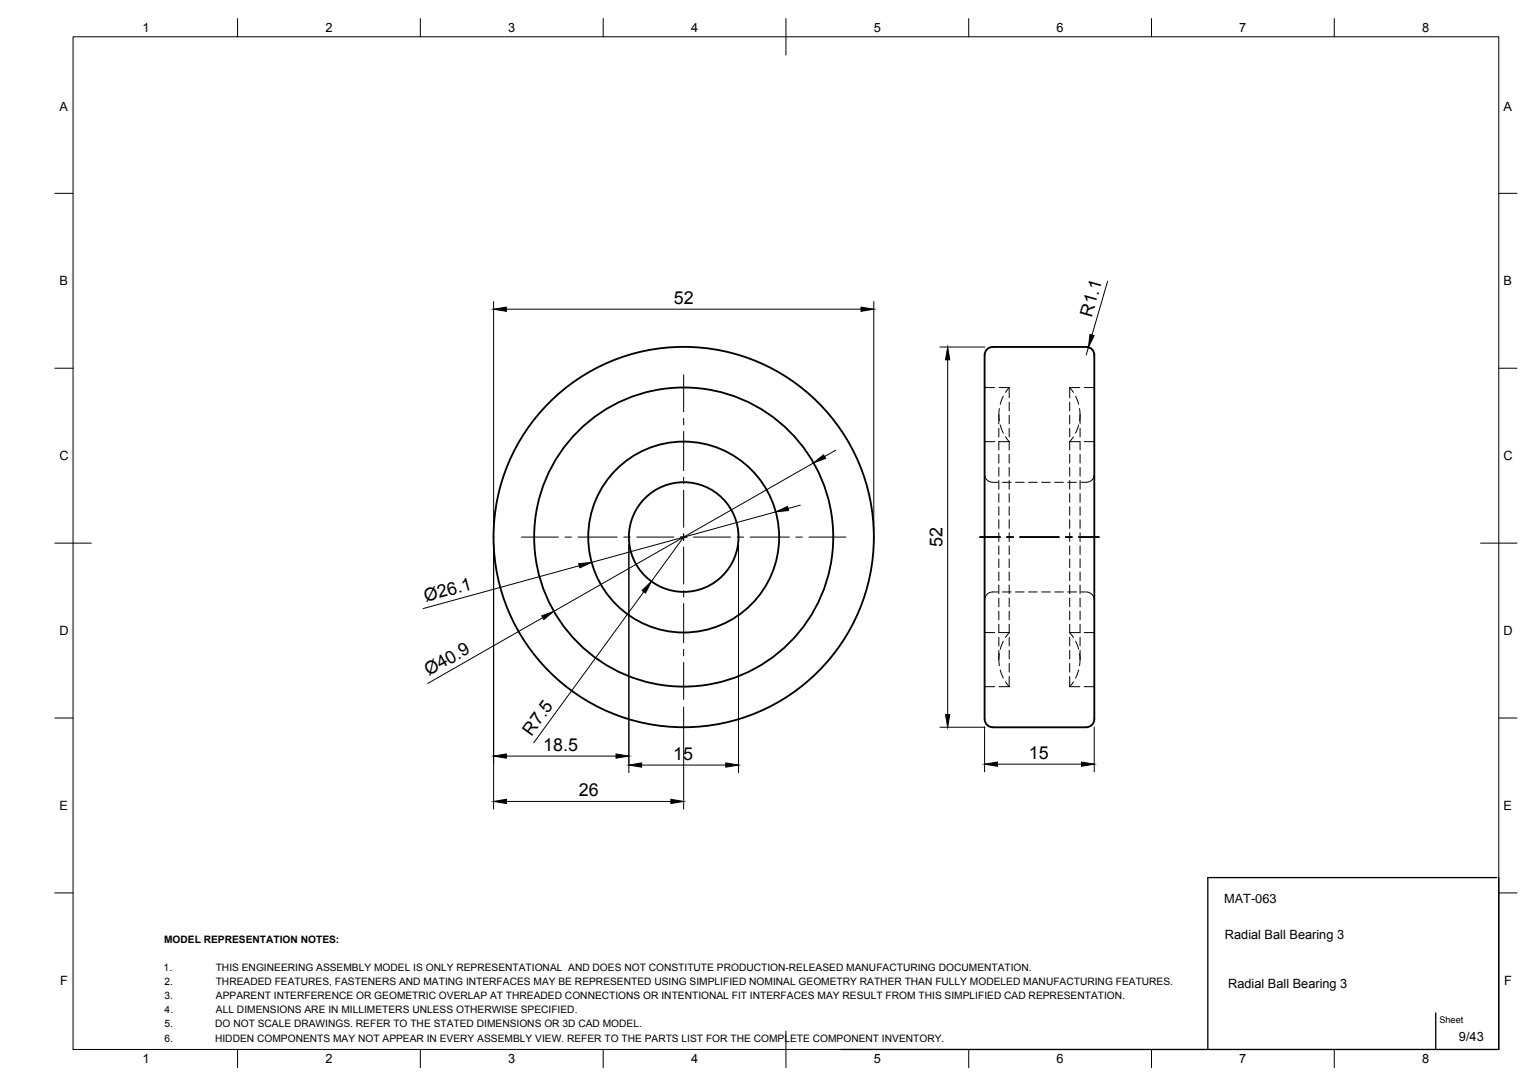
ISO-10303-21;
HEADER;
/* Generated by software containing ST-Developer
 * from STEP Tools, Inc. (www.steptools.com) 
 */

FILE_DESCRIPTION(
/* description */ (''),
/* implementation_level */ '2;1');

FILE_NAME(
/* name */ 'Radial Ball Bearing 3.step',
/* time_stamp */ '2026-10-24T09:43:01-07:00',
/* author */ (''),
/* organization */ (''),
/* preprocessor_version */ 'ST-DEVELOPER v20.2',
/* originating_system */ 'Autodesk Translation Framework v15.15.0.0',
/* authorisation */ '');

FILE_SCHEMA (('AUTOMOTIVE_DESIGN { 1 0 10303 214 3 1 1 }'));
ENDSEC;

DATA;
#10=MECHANICAL_DESIGN_GEOMETRIC_PRESENTATION_REPRESENTATION('',(#279),#11112);
#187=TOROIDAL_SURFACE('',#6680,0.0248999989285722,0.00110000131901909);
#188=TOROIDAL_SURFACE('',#6685,0.0248999989285722,0.00110000131901909);
#189=TOROIDAL_SURFACE('',#6693,0.0248999989285722,0.00110000131901911);
#190=TOROIDAL_SURFACE('',#6700,0.0248999989285722,0.00110000131901911);
#191=TOROIDAL_SURFACE('',#6704,0.01675,0.00555000054498457);
#192=TOROIDAL_SURFACE('',#6713,0.01675,0.00555000054498457);
#193=TOROIDAL_SURFACE('',#6722,0.00860000107142784,0.00110000131901912);
#194=TOROIDAL_SURFACE('',#6726,0.00860000107142784,0.00110000131901912);
#195=TOROIDAL_SURFACE('',#6734,0.00860000107142785,0.00110000131901912);
#196=TOROIDAL_SURFACE('',#6737,0.00860000107142785,0.00110000131901912);
#213=SHAPE_REPRESENTATION_RELATIONSHIP('SRR','None',#11236,#246);
#246=ADVANCED_BREP_SHAPE_REPRESENTATION('',(#312),#11081);
#279=STYLED_ITEM('',(#11425),#312);
#312=MANIFOLD_SOLID_BREP('Radial Ball Bearing 3',#6016);
#393=FACE_BOUND('',#1206,.T.);
#394=FACE_BOUND('',#1211,.T.);
#395=FACE_BOUND('',#1217,.T.);
#396=FACE_BOUND('',#1222,.T.);
#530=PLANE('',#6691);
#531=PLANE('',#6702);
#532=PLANE('',#6717);
#533=PLANE('',#6728);
#784=FACE_OUTER_BOUND('',#1202,.T.);
#785=FACE_OUTER_BOUND('',#1203,.T.);
#786=FACE_OUTER_BOUND('',#1204,.T.);
#787=FACE_OUTER_BOUND('',#1205,.T.);
#788=FACE_OUTER_BOUND('',#1207,.T.);
#789=FACE_OUTER_BOUND('',#1208,.T.);
#790=FACE_OUTER_BOUND('',#1209,.T.);
#791=FACE_OUTER_BOUND('',#1210,.T.);
#792=FACE_OUTER_BOUND('',#1212,.T.);
#793=FACE_OUTER_BOUND('',#1213,.T.);
#794=FACE_OUTER_BOUND('',#1214,.T.);
#795=FACE_OUTER_BOUND('',#1215,.T.);
#796=FACE_OUTER_BOUND('',#1216,.T.);
#797=FACE_OUTER_BOUND('',#1218,.T.);
#798=FACE_OUTER_BOUND('',#1219,.T.);
#799=FACE_OUTER_BOUND('',#1220,.T.);
#800=FACE_OUTER_BOUND('',#1221,.T.);
#801=FACE_OUTER_BOUND('',#1223,.T.);
#802=FACE_OUTER_BOUND('',#1224,.T.);
#803=FACE_OUTER_BOUND('',#1225,.T.);
#1202=EDGE_LOOP('',(#4431,#4432,#4433,#4434));
#1203=EDGE_LOOP('',(#4435,#4436,#4437,#4438));
#1204=EDGE_LOOP('',(#4439,#4440,#4441,#4442,#4443,#4444));
#1205=EDGE_LOOP('',(#4445,#4446));
#1206=EDGE_LOOP('',(#4447));
#1207=EDGE_LOOP('',(#4448,#4449,#4450,#4451));
#1208=EDGE_LOOP('',(#4452,#4453,#4454,#4455,#4456));
#1209=EDGE_LOOP('',(#4457,#4458,#4459,#4460));
#1210=EDGE_LOOP('',(#4461,#4462));
#1211=EDGE_LOOP('',(#4463));
#1212=EDGE_LOOP('',(#4464,#4465,#4466,#4467,#4468,#4469));
#1213=EDGE_LOOP('',(#4470,#4471,#4472,#4473,#4474));
#1214=EDGE_LOOP('',(#4475,#4476,#4477,#4478,#4479));
#1215=EDGE_LOOP('',(#4480,#4481,#4482,#4483,#4484,#4485));
#1216=EDGE_LOOP('',(#4486));
#1217=EDGE_LOOP('',(#4487,#4488));
#1218=EDGE_LOOP('',(#4489,#4490,#4491,#4492,#4493));
#1219=EDGE_LOOP('',(#4494,#4495,#4496,#4497));
#1220=EDGE_LOOP('',(#4498,#4499,#4500,#4501));
#1221=EDGE_LOOP('',(#4502));
#1222=EDGE_LOOP('',(#4503,#4504));
#1223=EDGE_LOOP('',(#4505,#4506,#4507,#4508,#4509,#4510));
#1224=EDGE_LOOP('',(#4511,#4512,#4513,#4514));
#1225=EDGE_LOOP('',(#4515,#4516,#4517,#4518));
#1643=LINE('',#9850,#2002);
#1644=LINE('',#9862,#2003);
#1645=LINE('',#9882,#2004);
#1646=LINE('',#9885,#2005);
#1647=LINE('',#9901,#2006);
#1648=LINE('',#9917,#2007);
#2002=VECTOR('',#7913,0.026);
#2003=VECTOR('',#7928,0.02045);
#2004=VECTOR('',#7955,0.02045);
#2005=VECTOR('',#7958,0.01305);
#2006=VECTOR('',#7979,0.01305);
#2007=VECTOR('',#8000,0.0075);
#2430=CIRCLE('',#6681,0.0248999997701383);
#2431=CIRCLE('',#6682,0.00110000131901909);
#2432=CIRCLE('',#6683,0.0260000002475909);
#2433=CIRCLE('',#6684,0.00110000131901909);
#2434=CIRCLE('',#6686,0.0248999997701383);
#2435=CIRCLE('',#6687,0.0260000002475909);
#2436=CIRCLE('',#6689,0.026);
#2437=CIRCLE('',#6690,0.026);
#2438=CIRCLE('',#6692,0.02045);
#2439=CIRCLE('',#6694,0.00110000131901911);
#2440=CIRCLE('',#6695,0.0248999997701383);
#2441=CIRCLE('',#6696,0.0011000013190191);
#2442=CIRCLE('',#6698,0.02045);
#2443=CIRCLE('',#6699,0.02045);
#2444=CIRCLE('',#6701,0.0248999997701383);
#2445=CIRCLE('',#6703,0.02045);
#2446=CIRCLE('',#6705,0.00555000054498457);
#2447=CIRCLE('',#6706,0.0130499999271107);
#2448=CIRCLE('',#6707,0.0130499999271107);
#2449=CIRCLE('',#6709,0.02045);
#2450=CIRCLE('',#6710,0.02045);
#2451=CIRCLE('',#6712,0.01305);
#2452=CIRCLE('',#6714,0.01305);
#2453=CIRCLE('',#6715,0.00555000054498457);
#2454=CIRCLE('',#6716,0.01305);
#2455=CIRCLE('',#6718,0.00860000022986177);
#2456=CIRCLE('',#6719,0.00860000022986177);
#2457=CIRCLE('',#6721,0.01305);
#2458=CIRCLE('',#6723,0.00110000131901912);
#2459=CIRCLE('',#6724,0.00749999975240907);
#2460=CIRCLE('',#6725,0.00110000131901912);
#2461=CIRCLE('',#6727,0.00749999975240873);
#2462=CIRCLE('',#6729,0.00860000022986177);
#2463=CIRCLE('',#6730,0.00860000022986177);
#2464=CIRCLE('',#6732,0.0075);
#2465=CIRCLE('',#6733,0.00749999975240873);
#2466=CIRCLE('',#6735,0.00110000131901912);
#2467=CIRCLE('',#6736,0.00110000131901912);
#2832=VERTEX_POINT('',#9834);
#2833=VERTEX_POINT('',#9835);
#2834=VERTEX_POINT('',#9837);
#2835=VERTEX_POINT('',#9839);
#2836=VERTEX_POINT('',#9846);
#2837=VERTEX_POINT('',#9847);
#2838=VERTEX_POINT('',#9852);
#2839=VERTEX_POINT('',#9855);
#2840=VERTEX_POINT('',#9857);
#2841=VERTEX_POINT('',#9861);
#2842=VERTEX_POINT('',#9863);
#2843=VERTEX_POINT('',#9869);
#2844=VERTEX_POINT('',#9872);
#2845=VERTEX_POINT('',#9874);
#2846=VERTEX_POINT('',#9878);
#2847=VERTEX_POINT('',#9879);
#2848=VERTEX_POINT('',#9884);
#2849=VERTEX_POINT('',#9888);
#2850=VERTEX_POINT('',#9889);
#2851=VERTEX_POINT('',#9894);
#2852=VERTEX_POINT('',#9895);
#2853=VERTEX_POINT('',#9899);
#2854=VERTEX_POINT('',#9903);
#2855=VERTEX_POINT('',#9905);
#2856=VERTEX_POINT('',#9911);
#2857=VERTEX_POINT('',#9912);
#2858=VERTEX_POINT('',#9916);
#2859=VERTEX_POINT('',#9918);
#3419=EDGE_CURVE('',#2832,#2833,#2430,.T.);
#3420=EDGE_CURVE('',#2833,#2834,#2431,.T.);
#3421=EDGE_CURVE('',#2834,#2835,#2432,.F.);
#3422=EDGE_CURVE('',#2835,#2832,#2433,.T.);
#3423=EDGE_CURVE('',#2833,#2832,#2434,.T.);
#3424=EDGE_CURVE('',#2835,#2834,#2435,.T.);
#3425=EDGE_CURVE('',#2836,#2837,#2436,.F.);
#3426=EDGE_CURVE('',#2837,#2836,#2437,.F.);
#3427=EDGE_CURVE('',#2836,#2834,#1643,.T.);
#3428=EDGE_CURVE('',#2838,#2838,#2438,.T.);
#3429=EDGE_CURVE('',#2836,#2839,#2439,.T.);
#3430=EDGE_CURVE('',#2839,#2840,#2440,.F.);
#3431=EDGE_CURVE('',#2840,#2837,#2441,.T.);
#3432=EDGE_CURVE('',#2838,#2841,#1644,.T.);
#3433=EDGE_CURVE('',#2842,#2841,#2442,.F.);
#3434=EDGE_CURVE('',#2841,#2842,#2443,.F.);
#3435=EDGE_CURVE('',#2840,#2839,#2444,.F.);
#3436=EDGE_CURVE('',#2843,#2843,#2445,.F.);
#3437=EDGE_CURVE('',#2842,#2844,#2446,.T.);
#3438=EDGE_CURVE('',#2844,#2845,#2447,.T.);
#3439=EDGE_CURVE('',#2845,#2844,#2448,.T.);
#3440=EDGE_CURVE('',#2846,#2847,#2449,.F.);
#3441=EDGE_CURVE('',#2847,#2846,#2450,.F.);
#3442=EDGE_CURVE('',#2847,#2843,#1645,.T.);
#3443=EDGE_CURVE('',#2845,#2848,#1646,.T.);
#3444=EDGE_CURVE('',#2848,#2848,#2451,.T.);
#3445=EDGE_CURVE('',#2849,#2850,#2452,.T.);
#3446=EDGE_CURVE('',#2850,#2846,#2453,.T.);
#3447=EDGE_CURVE('',#2850,#2849,#2454,.T.);
#3448=EDGE_CURVE('',#2851,#2852,#2455,.T.);
#3449=EDGE_CURVE('',#2852,#2851,#2456,.T.);
#3450=EDGE_CURVE('',#2853,#2853,#2457,.F.);
#3451=EDGE_CURVE('',#2853,#2849,#1647,.T.);
#3452=EDGE_CURVE('',#2852,#2854,#2458,.T.);
#3453=EDGE_CURVE('',#2854,#2855,#2459,.T.);
#3454=EDGE_CURVE('',#2855,#2851,#2460,.T.);
#3455=EDGE_CURVE('',#2855,#2854,#2461,.T.);
#3456=EDGE_CURVE('',#2856,#2857,#2462,.F.);
#3457=EDGE_CURVE('',#2857,#2856,#2463,.F.);
#3458=EDGE_CURVE('',#2854,#2858,#1648,.T.);
#3459=EDGE_CURVE('',#2859,#2858,#2464,.F.);
#3460=EDGE_CURVE('',#2858,#2859,#2465,.F.);
#3461=EDGE_CURVE('',#2858,#2856,#2466,.T.);
#3462=EDGE_CURVE('',#2857,#2859,#2467,.T.);
#4431=ORIENTED_EDGE('',*,*,#3419,.T.);
#4432=ORIENTED_EDGE('',*,*,#3420,.T.);
#4433=ORIENTED_EDGE('',*,*,#3421,.T.);
#4434=ORIENTED_EDGE('',*,*,#3422,.T.);
#4435=ORIENTED_EDGE('',*,*,#3420,.F.);
#4436=ORIENTED_EDGE('',*,*,#3423,.T.);
#4437=ORIENTED_EDGE('',*,*,#3422,.F.);
#4438=ORIENTED_EDGE('',*,*,#3424,.T.);
#4439=ORIENTED_EDGE('',*,*,#3425,.T.);
#4440=ORIENTED_EDGE('',*,*,#3426,.T.);
#4441=ORIENTED_EDGE('',*,*,#3427,.T.);
#4442=ORIENTED_EDGE('',*,*,#3424,.F.);
#4443=ORIENTED_EDGE('',*,*,#3421,.F.);
#4444=ORIENTED_EDGE('',*,*,#3427,.F.);
#4445=ORIENTED_EDGE('',*,*,#3419,.F.);
#4446=ORIENTED_EDGE('',*,*,#3423,.F.);
#4447=ORIENTED_EDGE('',*,*,#3428,.T.);
#4448=ORIENTED_EDGE('',*,*,#3425,.F.);
#4449=ORIENTED_EDGE('',*,*,#3429,.T.);
#4450=ORIENTED_EDGE('',*,*,#3430,.T.);
#4451=ORIENTED_EDGE('',*,*,#3431,.T.);
#4452=ORIENTED_EDGE('',*,*,#3428,.F.);
#4453=ORIENTED_EDGE('',*,*,#3432,.T.);
#4454=ORIENTED_EDGE('',*,*,#3433,.F.);
#4455=ORIENTED_EDGE('',*,*,#3434,.F.);
#4456=ORIENTED_EDGE('',*,*,#3432,.F.);
#4457=ORIENTED_EDGE('',*,*,#3429,.F.);
#4458=ORIENTED_EDGE('',*,*,#3426,.F.);
#4459=ORIENTED_EDGE('',*,*,#3431,.F.);
#4460=ORIENTED_EDGE('',*,*,#3435,.T.);
#4461=ORIENTED_EDGE('',*,*,#3430,.F.);
#4462=ORIENTED_EDGE('',*,*,#3435,.F.);
#4463=ORIENTED_EDGE('',*,*,#3436,.T.);
#4464=ORIENTED_EDGE('',*,*,#3434,.T.);
#4465=ORIENTED_EDGE('',*,*,#3437,.T.);
#4466=ORIENTED_EDGE('',*,*,#3438,.T.);
#4467=ORIENTED_EDGE('',*,*,#3439,.T.);
#4468=ORIENTED_EDGE('',*,*,#3437,.F.);
#4469=ORIENTED_EDGE('',*,*,#3433,.T.);
#4470=ORIENTED_EDGE('',*,*,#3440,.F.);
#4471=ORIENTED_EDGE('',*,*,#3441,.F.);
#4472=ORIENTED_EDGE('',*,*,#3442,.T.);
#4473=ORIENTED_EDGE('',*,*,#3436,.F.);
#4474=ORIENTED_EDGE('',*,*,#3442,.F.);
#4475=ORIENTED_EDGE('',*,*,#3439,.F.);
#4476=ORIENTED_EDGE('',*,*,#3443,.T.);
#4477=ORIENTED_EDGE('',*,*,#3444,.T.);
#4478=ORIENTED_EDGE('',*,*,#3443,.F.);
#4479=ORIENTED_EDGE('',*,*,#3438,.F.);
#4480=ORIENTED_EDGE('',*,*,#3445,.T.);
#4481=ORIENTED_EDGE('',*,*,#3446,.T.);
#4482=ORIENTED_EDGE('',*,*,#3440,.T.);
#4483=ORIENTED_EDGE('',*,*,#3441,.T.);
#4484=ORIENTED_EDGE('',*,*,#3446,.F.);
#4485=ORIENTED_EDGE('',*,*,#3447,.T.);
#4486=ORIENTED_EDGE('',*,*,#3444,.F.);
#4487=ORIENTED_EDGE('',*,*,#3448,.T.);
#4488=ORIENTED_EDGE('',*,*,#3449,.T.);
#4489=ORIENTED_EDGE('',*,*,#3450,.T.);
#4490=ORIENTED_EDGE('',*,*,#3451,.T.);
#4491=ORIENTED_EDGE('',*,*,#3447,.F.);
#4492=ORIENTED_EDGE('',*,*,#3445,.F.);
#4493=ORIENTED_EDGE('',*,*,#3451,.F.);
#4494=ORIENTED_EDGE('',*,*,#3452,.T.);
#4495=ORIENTED_EDGE('',*,*,#3453,.T.);
#4496=ORIENTED_EDGE('',*,*,#3454,.T.);
#4497=ORIENTED_EDGE('',*,*,#3449,.F.);
#4498=ORIENTED_EDGE('',*,*,#3455,.T.);
#4499=ORIENTED_EDGE('',*,*,#3452,.F.);
#4500=ORIENTED_EDGE('',*,*,#3448,.F.);
#4501=ORIENTED_EDGE('',*,*,#3454,.F.);
#4502=ORIENTED_EDGE('',*,*,#3450,.F.);
#4503=ORIENTED_EDGE('',*,*,#3456,.T.);
#4504=ORIENTED_EDGE('',*,*,#3457,.T.);
#4505=ORIENTED_EDGE('',*,*,#3453,.F.);
#4506=ORIENTED_EDGE('',*,*,#3458,.T.);
#4507=ORIENTED_EDGE('',*,*,#3459,.F.);
#4508=ORIENTED_EDGE('',*,*,#3460,.F.);
#4509=ORIENTED_EDGE('',*,*,#3458,.F.);
#4510=ORIENTED_EDGE('',*,*,#3455,.F.);
#4511=ORIENTED_EDGE('',*,*,#3461,.T.);
#4512=ORIENTED_EDGE('',*,*,#3457,.F.);
#4513=ORIENTED_EDGE('',*,*,#3462,.T.);
#4514=ORIENTED_EDGE('',*,*,#3459,.T.);
#4515=ORIENTED_EDGE('',*,*,#3456,.F.);
#4516=ORIENTED_EDGE('',*,*,#3461,.F.);
#4517=ORIENTED_EDGE('',*,*,#3460,.T.);
#4518=ORIENTED_EDGE('',*,*,#3462,.F.);
#5548=CYLINDRICAL_SURFACE('',#6688,0.026);
#5549=CYLINDRICAL_SURFACE('',#6697,0.02045);
#5550=CYLINDRICAL_SURFACE('',#6708,0.02045);
#5551=CYLINDRICAL_SURFACE('',#6711,0.01305);
#5552=CYLINDRICAL_SURFACE('',#6720,0.01305);
#5553=CYLINDRICAL_SURFACE('',#6731,0.0075);
#5757=ADVANCED_FACE('',(#784),#187,.T.);
#5758=ADVANCED_FACE('',(#785),#188,.T.);
#5759=ADVANCED_FACE('',(#786),#5548,.T.);
#5760=ADVANCED_FACE('',(#787,#393),#530,.T.);
#5761=ADVANCED_FACE('',(#788),#189,.T.);
#5762=ADVANCED_FACE('',(#789),#5549,.F.);
#5763=ADVANCED_FACE('',(#790),#190,.T.);
#5764=ADVANCED_FACE('',(#791,#394),#531,.T.);
#5765=ADVANCED_FACE('',(#792),#191,.T.);
#5766=ADVANCED_FACE('',(#793),#5550,.F.);
#5767=ADVANCED_FACE('',(#794),#5551,.T.);
#5768=ADVANCED_FACE('',(#795),#192,.T.);
#5769=ADVANCED_FACE('',(#796,#395),#532,.T.);
#5770=ADVANCED_FACE('',(#797),#5552,.T.);
#5771=ADVANCED_FACE('',(#798),#193,.T.);
#5772=ADVANCED_FACE('',(#799),#194,.T.);
#5773=ADVANCED_FACE('',(#800,#396),#533,.T.);
#5774=ADVANCED_FACE('',(#801),#5553,.F.);
#5775=ADVANCED_FACE('',(#802),#195,.T.);
#5776=ADVANCED_FACE('',(#803),#196,.T.);
#6016=CLOSED_SHELL('',(#5757,#5758,#5759,#5760,#5761,#5762,#5763,#5764,
#5765,#5766,#5767,#5768,#5769,#5770,#5771,#5772,#5773,#5774,#5775,#5776));
#6679=AXIS2_PLACEMENT_3D('',#9832,#7889,#7890);
#6680=AXIS2_PLACEMENT_3D('',#9833,#7891,#7892);
#6681=AXIS2_PLACEMENT_3D('',#9836,#7893,#7894);
#6682=AXIS2_PLACEMENT_3D('',#9838,#7895,#7896);
#6683=AXIS2_PLACEMENT_3D('',#9840,#7897,#7898);
#6684=AXIS2_PLACEMENT_3D('',#9841,#7899,#7900);
#6685=AXIS2_PLACEMENT_3D('',#9842,#7901,#7902);
#6686=AXIS2_PLACEMENT_3D('',#9843,#7903,#7904);
#6687=AXIS2_PLACEMENT_3D('',#9844,#7905,#7906);
#6688=AXIS2_PLACEMENT_3D('',#9845,#7907,#7908);
#6689=AXIS2_PLACEMENT_3D('',#9848,#7909,#7910);
#6690=AXIS2_PLACEMENT_3D('',#9849,#7911,#7912);
#6691=AXIS2_PLACEMENT_3D('',#9851,#7914,#7915);
#6692=AXIS2_PLACEMENT_3D('',#9853,#7916,#7917);
#6693=AXIS2_PLACEMENT_3D('',#9854,#7918,#7919);
#6694=AXIS2_PLACEMENT_3D('',#9856,#7920,#7921);
#6695=AXIS2_PLACEMENT_3D('',#9858,#7922,#7923);
#6696=AXIS2_PLACEMENT_3D('',#9859,#7924,#7925);
#6697=AXIS2_PLACEMENT_3D('',#9860,#7926,#7927);
#6698=AXIS2_PLACEMENT_3D('',#9864,#7929,#7930);
#6699=AXIS2_PLACEMENT_3D('',#9865,#7931,#7932);
#6700=AXIS2_PLACEMENT_3D('',#9866,#7933,#7934);
#6701=AXIS2_PLACEMENT_3D('',#9867,#7935,#7936);
#6702=AXIS2_PLACEMENT_3D('',#9868,#7937,#7938);
#6703=AXIS2_PLACEMENT_3D('',#9870,#7939,#7940);
#6704=AXIS2_PLACEMENT_3D('',#9871,#7941,#7942);
#6705=AXIS2_PLACEMENT_3D('',#9873,#7943,#7944);
#6706=AXIS2_PLACEMENT_3D('',#9875,#7945,#7946);
#6707=AXIS2_PLACEMENT_3D('',#9876,#7947,#7948);
#6708=AXIS2_PLACEMENT_3D('',#9877,#7949,#7950);
#6709=AXIS2_PLACEMENT_3D('',#9880,#7951,#7952);
#6710=AXIS2_PLACEMENT_3D('',#9881,#7953,#7954);
#6711=AXIS2_PLACEMENT_3D('',#9883,#7956,#7957);
#6712=AXIS2_PLACEMENT_3D('',#9886,#7959,#7960);
#6713=AXIS2_PLACEMENT_3D('',#9887,#7961,#7962);
#6714=AXIS2_PLACEMENT_3D('',#9890,#7963,#7964);
#6715=AXIS2_PLACEMENT_3D('',#9891,#7965,#7966);
#6716=AXIS2_PLACEMENT_3D('',#9892,#7967,#7968);
#6717=AXIS2_PLACEMENT_3D('',#9893,#7969,#7970);
#6718=AXIS2_PLACEMENT_3D('',#9896,#7971,#7972);
#6719=AXIS2_PLACEMENT_3D('',#9897,#7973,#7974);
#6720=AXIS2_PLACEMENT_3D('',#9898,#7975,#7976);
#6721=AXIS2_PLACEMENT_3D('',#9900,#7977,#7978);
#6722=AXIS2_PLACEMENT_3D('',#9902,#7980,#7981);
#6723=AXIS2_PLACEMENT_3D('',#9904,#7982,#7983);
#6724=AXIS2_PLACEMENT_3D('',#9906,#7984,#7985);
#6725=AXIS2_PLACEMENT_3D('',#9907,#7986,#7987);
#6726=AXIS2_PLACEMENT_3D('',#9908,#7988,#7989);
#6727=AXIS2_PLACEMENT_3D('',#9909,#7990,#7991);
#6728=AXIS2_PLACEMENT_3D('',#9910,#7992,#7993);
#6729=AXIS2_PLACEMENT_3D('',#9913,#7994,#7995);
#6730=AXIS2_PLACEMENT_3D('',#9914,#7996,#7997);
#6731=AXIS2_PLACEMENT_3D('',#9915,#7998,#7999);
#6732=AXIS2_PLACEMENT_3D('',#9919,#8001,#8002);
#6733=AXIS2_PLACEMENT_3D('',#9920,#8003,#8004);
#6734=AXIS2_PLACEMENT_3D('',#9921,#8005,#8006);
#6735=AXIS2_PLACEMENT_3D('',#9922,#8007,#8008);
#6736=AXIS2_PLACEMENT_3D('',#9923,#8009,#8010);
#6737=AXIS2_PLACEMENT_3D('',#9924,#8011,#8012);
#7889=DIRECTION('axis',(0.,0.,1.));
#7890=DIRECTION('refdir',(1.,0.,0.));
#7891=DIRECTION('center_axis',(1.,4.17203717831812E-9,1.01277540341552E-17));
#7892=DIRECTION('ref_axis',(-4.1720371751696E-9,1.,0.));
#7893=DIRECTION('center_axis',(1.,4.17203717831812E-9,1.01277540341552E-17));
#7894=DIRECTION('ref_axis',(-4.17203717831812E-9,1.,-1.69634196247466E-42));
#7895=DIRECTION('center_axis',(8.36866394062756E-10,1.,-8.36884415538179E-10));
#7896=DIRECTION('ref_axis',(-7.96162761077703E-7,8.36885081819775E-10,0.999999999999683));
#7897=DIRECTION('center_axis',(1.,4.17203717831812E-9,1.01277540341552E-17));
#7898=DIRECTION('ref_axis',(-4.17203717831812E-9,1.,-1.69634196247466E-42));
#7899=DIRECTION('center_axis',(8.36869948186391E-10,1.,8.36891441629708E-10));
#7900=DIRECTION('ref_axis',(-0.999999999999707,8.36870588457614E-10,-7.65059166582913E-7));
#7901=DIRECTION('center_axis',(1.,-4.17203708245403E-9,6.73890284431642E-18));
#7902=DIRECTION('ref_axis',(-4.1720370750894E-9,-1.,5.66553889764798E-16));
#7903=DIRECTION('center_axis',(1.,-4.17203708245403E-9,6.73890284431642E-18));
#7904=DIRECTION('ref_axis',(4.17203708245403E-9,1.,-1.23465054354127E-43));
#7905=DIRECTION('center_axis',(-1.,4.17203697154146E-9,4.27849718847752E-19));
#7906=DIRECTION('ref_axis',(-4.27008851558771E-17,-5.34839554841822E-9,
1.));
#7907=DIRECTION('center_axis',(1.,0.,-3.33600668457079E-17));
#7908=DIRECTION('ref_axis',(-3.33600668457079E-17,0.,-1.));
#7909=DIRECTION('center_axis',(1.,0.,-3.33600668457079E-17));
#7910=DIRECTION('ref_axis',(-3.33600668457079E-17,0.,-1.));
#7911=DIRECTION('center_axis',(1.,0.,0.));
#7912=DIRECTION('ref_axis',(0.,-4.64793894161955E-10,-1.));
#7913=DIRECTION('',(-1.,0.,3.33600668457079E-17));
#7914=DIRECTION('center_axis',(-1.,1.53144334479515E-17,1.9842828066192E-17));
#7915=DIRECTION('ref_axis',(1.9842828066192E-17,0.,1.));
#7916=DIRECTION('center_axis',(1.,0.,0.));
#7917=DIRECTION('ref_axis',(0.,0.,-1.));
#7918=DIRECTION('center_axis',(1.,-4.17203727418451E-9,-1.07069540457721E-17));
#7919=DIRECTION('ref_axis',(4.1720372752498E-9,1.,0.));
#7920=DIRECTION('center_axis',(-8.36866342496331E-10,1.,-8.36883936494317E-10));
#7921=DIRECTION('ref_axis',(0.999999999999707,8.36866982761818E-10,7.65059174657239E-7));
#7922=DIRECTION('center_axis',(1.,-4.17203727418451E-9,-1.07069540457721E-17));
#7923=DIRECTION('ref_axis',(4.17203727418451E-9,1.,1.45967462857766E-42));
#7924=DIRECTION('center_axis',(-8.36844869453255E-10,1.,8.36865935422119E-10));
#7925=DIRECTION('ref_axis',(9.00645352209864E-7,8.36866689122222E-10,-0.999999999999595));
#7926=DIRECTION('center_axis',(1.,0.,0.));
#7927=DIRECTION('ref_axis',(0.,0.,-1.));
#7928=DIRECTION('',(1.,0.,0.));
#7929=DIRECTION('center_axis',(1.,0.,0.));
#7930=DIRECTION('ref_axis',(0.,-4.29586394988857E-10,-1.));
#7931=DIRECTION('center_axis',(1.,0.,0.));
#7932=DIRECTION('ref_axis',(0.,-4.29586394988857E-10,-1.));
#7933=DIRECTION('center_axis',(1.,4.17203725971588E-9,2.0031116033889E-18));
#7934=DIRECTION('ref_axis',(4.1720372752498E-9,-1.,5.66553889764798E-16));
#7935=DIRECTION('center_axis',(1.,4.17203725971588E-9,2.0031116033889E-18));
#7936=DIRECTION('ref_axis',(-4.17203725971588E-9,1.,5.39459847610519E-43));
#7937=DIRECTION('center_axis',(1.,1.53144334479515E-17,-1.9842828066192E-17));
#7938=DIRECTION('ref_axis',(-1.9842828066192E-17,0.,-1.));
#7939=DIRECTION('center_axis',(1.,0.,0.));
#7940=DIRECTION('ref_axis',(0.,0.,-1.));
#7941=DIRECTION('center_axis',(1.,6.36556116938371E-17,1.00386354793954E-17));
#7942=DIRECTION('ref_axis',(-6.3655612933414E-17,1.,0.));
#7943=DIRECTION('center_axis',(1.00386354793954E-17,1.22464679914735E-16,
-1.));
#7944=DIRECTION('ref_axis',(6.36556105223495E-17,-1.,-1.22464679914735E-16));
#7945=DIRECTION('center_axis',(1.,1.35504238326755E-16,2.34999225611352E-17));
#7946=DIRECTION('ref_axis',(-1.35504238326755E-16,1.,1.40763492406121E-49));
#7947=DIRECTION('center_axis',(1.,1.35504238326755E-16,2.34999225611352E-17));
#7948=DIRECTION('ref_axis',(-1.35504238326755E-16,1.,1.40763492406121E-49));
#7949=DIRECTION('center_axis',(1.,0.,0.));
#7950=DIRECTION('ref_axis',(0.,0.,-1.));
#7951=DIRECTION('center_axis',(-1.,0.,0.));
#7952=DIRECTION('ref_axis',(0.,-6.60206605267583E-10,1.));
#7953=DIRECTION('center_axis',(-1.,0.,0.));
#7954=DIRECTION('ref_axis',(0.,-6.60206605267583E-10,1.));
#7955=DIRECTION('',(1.,0.,0.));
#7956=DIRECTION('center_axis',(1.,0.,0.));
#7957=DIRECTION('ref_axis',(0.,0.,-1.));
#7958=DIRECTION('',(-1.,0.,0.));
#7959=DIRECTION('center_axis',(1.,0.,0.));
#7960=DIRECTION('ref_axis',(0.,0.,-1.));
#7961=DIRECTION('center_axis',(1.,1.18552772674719E-16,-1.97711088800387E-17));
#7962=DIRECTION('ref_axis',(-1.18552772074394E-16,1.,0.));
#7963=DIRECTION('center_axis',(-1.,0.,0.));
#7964=DIRECTION('ref_axis',(0.,-2.05103586755523E-10,1.));
#7965=DIRECTION('center_axis',(-1.97711088800387E-17,1.22464679914735E-16,
-1.));
#7966=DIRECTION('ref_axis',(1.18552771796194E-16,-1.,-1.22464679914735E-16));
#7967=DIRECTION('center_axis',(-1.,0.,0.));
#7968=DIRECTION('ref_axis',(0.,-2.05103586755523E-10,1.));
#7969=DIRECTION('center_axis',(-1.,2.92206431305708E-17,3.78610282642285E-17));
#7970=DIRECTION('ref_axis',(3.78610282642285E-17,0.,1.));
#7971=DIRECTION('center_axis',(1.,1.20795004338275E-8,6.525328094131E-17));
#7972=DIRECTION('ref_axis',(-1.20795004338275E-8,1.,4.44135209129409E-41));
#7973=DIRECTION('center_axis',(1.,-1.20794999078492E-8,-6.65136044666218E-17));
#7974=DIRECTION('ref_axis',(1.20794999078492E-8,1.,-3.20659696454606E-41));
#7975=DIRECTION('center_axis',(1.,0.,0.));
#7976=DIRECTION('ref_axis',(0.,0.,-1.));
#7977=DIRECTION('center_axis',(1.,0.,0.));
#7978=DIRECTION('ref_axis',(0.,0.,-1.));
#7979=DIRECTION('',(-1.,0.,0.));
#7980=DIRECTION('center_axis',(1.,-1.20794999078492E-8,-6.65136044666218E-17));
#7981=DIRECTION('ref_axis',(-1.20794999243885E-8,-1.,-5.21792575105832E-12));
#7982=DIRECTION('center_axis',(-3.90112644891662E-10,-1.,-3.90117034748036E-10));
#7983=DIRECTION('ref_axis',(-7.96162782272821E-7,3.90117345341081E-10,-0.999999999999683));
#7984=DIRECTION('center_axis',(1.,-1.20794992145421E-8,-4.8381018443521E-19));
#7985=DIRECTION('ref_axis',(1.48029741503464E-16,1.78300800621899E-8,-1.));
#7986=DIRECTION('center_axis',(-3.90083830404282E-10,-1.,3.90119162273478E-10));
#7987=DIRECTION('ref_axis',(-0.999999999999707,3.90084128868405E-10,7.65059156489968E-7));
#7988=DIRECTION('center_axis',(1.,1.20795004338275E-8,6.525328094131E-17));
#7989=DIRECTION('ref_axis',(-1.20795004609008E-8,1.,0.));
#7990=DIRECTION('center_axis',(1.,1.20795004338275E-8,6.525328094131E-17));
#7991=DIRECTION('ref_axis',(-1.20795004338275E-8,1.,4.44135209129409E-41));
#7992=DIRECTION('center_axis',(1.,2.92206431305708E-17,-3.78610282642285E-17));
#7993=DIRECTION('ref_axis',(-3.78610282642285E-17,0.,-1.));
#7994=DIRECTION('center_axis',(1.,-1.20794999071527E-8,2.28224857621035E-17));
#7995=DIRECTION('ref_axis',(1.20794999071527E-8,1.,-1.89856639006012E-41));
#7996=DIRECTION('center_axis',(1.,1.20794999172425E-8,-1.59545740616835E-17));
#7997=DIRECTION('ref_axis',(-1.20794999172425E-8,1.,2.99570552288603E-42));
#7998=DIRECTION('center_axis',(1.,0.,-1.15648231731787E-16));
#7999=DIRECTION('ref_axis',(-1.15648231731787E-16,0.,-1.));
#8000=DIRECTION('',(1.,0.,-1.15648231731787E-16));
#8001=DIRECTION('center_axis',(1.,0.,0.));
#8002=DIRECTION('ref_axis',(0.,-4.29586131949163E-10,-1.));
#8003=DIRECTION('center_axis',(1.,-1.20794999071527E-8,2.28224857621035E-17));
#8004=DIRECTION('ref_axis',(1.20794999071527E-8,1.,-1.89856639006012E-41));
#8005=DIRECTION('center_axis',(1.,1.20794999172425E-8,-1.59545740616835E-17));
#8006=DIRECTION('ref_axis',(1.20794999243885E-8,-1.,-8.2319592183107E-12));
#8007=DIRECTION('center_axis',(3.9010897446429E-10,-1.,-3.90108144056802E-10));
#8008=DIRECTION('ref_axis',(0.999999999999707,3.90109272919983E-10,-7.65059154471383E-7));
#8009=DIRECTION('center_axis',(3.90083837031876E-10,-1.,3.90119162425402E-10));
#8010=DIRECTION('ref_axis',(7.96162783282112E-7,3.90119472995512E-10,0.999999999999683));
#8011=DIRECTION('center_axis',(1.,-1.20794999071527E-8,2.28224857621035E-17));
#8012=DIRECTION('ref_axis',(1.20794999243885E-8,1.,0.));
#9832=CARTESIAN_POINT('',(0.,0.,0.));
#9833=CARTESIAN_POINT('Origin',(-0.00639999889435817,-1.33725586897056E-10,
-2.60202312123977E-18));
#9834=CARTESIAN_POINT('',(-0.00750000021337694,-2.62982038223811E-17,-0.0248999997701383));
#9835=CARTESIAN_POINT('',(-0.00750000021337694,-9.33158505355009E-18,0.0248999997701383));
#9836=CARTESIAN_POINT('Origin',(-0.00750000021337694,-1.38314833296201E-10,
-2.61316366403604E-18));
#9837=CARTESIAN_POINT('',(-0.00639999976976533,-1.58005919577827E-12,0.0260000002475909));
#9838=CARTESIAN_POINT('Origin',(-0.00639999889435817,-9.20581548326642E-13,
0.0248999989285722));
#9839=CARTESIAN_POINT('',(-0.00639999976976533,-3.35121902792442E-17,-0.0260000002475909));
#9840=CARTESIAN_POINT('Origin',(-0.00639999977013826,-1.33725590550843E-10,
-2.60202313010945E-18));
#9841=CARTESIAN_POINT('Origin',(-0.00639999889435817,-9.20629689158185E-13,
-0.0248999989285722));
#9842=CARTESIAN_POINT('Origin',(-0.00639999889435817,1.33725588194013E-10,
-2.25687613815873E-19));
#9843=CARTESIAN_POINT('Origin',(-0.00750000021337694,1.38314834487708E-10,
-2.3310041583336E-19));
#9844=CARTESIAN_POINT('Origin',(-0.00639999977013826,1.3372558821988E-10,
4.44089209850063E-18));
#9845=CARTESIAN_POINT('Origin',(-0.0206375,0.,-4.33144407778805E-52));
#9846=CARTESIAN_POINT('',(0.00639999998722997,-6.70342338705283E-12,0.0260000000825303));
#9847=CARTESIAN_POINT('',(0.00639999998722997,-5.37097589710219E-12,-0.0260000000825303));
#9848=CARTESIAN_POINT('Origin',(0.0064,0.,-9.01972807340825E-19));
#9849=CARTESIAN_POINT('Origin',(0.0064,2.91826343292479E-18,0.));
#9850=CARTESIAN_POINT('',(-0.0206375,-3.18408167778312E-18,0.026));
#9851=CARTESIAN_POINT('Origin',(-0.0075,-1.31838984174237E-18,-1.2490009027033E-18));
#9852=CARTESIAN_POINT('',(-0.0075,-2.50440270425634E-18,0.02045));
#9853=CARTESIAN_POINT('Origin',(-0.0075,0.,0.));
#9854=CARTESIAN_POINT('Origin',(0.00639999889435816,-1.33725593635445E-10,
-3.59711256079879E-19));
#9855=CARTESIAN_POINT('',(0.00750000021337694,-1.05191955076574E-17,0.0248999997701383));
#9856=CARTESIAN_POINT('Origin',(0.00639999889435816,-9.20588335445364E-13,
0.0248999989285722));
#9857=CARTESIAN_POINT('',(0.00750000021337694,-2.93287844693988E-17,-0.0248999997701383));
#9858=CARTESIAN_POINT('Origin',(0.00750000021337694,-1.38314840140043E-10,
-3.71488919652902E-19));
#9859=CARTESIAN_POINT('Origin',(0.00639999889435816,-9.20608946339399E-13,
-0.0248999989285722));
#9860=CARTESIAN_POINT('Origin',(-0.0206375,0.,0.));
#9861=CARTESIAN_POINT('',(-0.00413672599961696,1.0458235455062E-18,0.0204500000364447));
#9862=CARTESIAN_POINT('',(-0.0206375,-2.50440270425634E-18,0.02045));
#9863=CARTESIAN_POINT('',(-0.004136726,-0.02045,-2.79956704802153E-18));
#9864=CARTESIAN_POINT('Origin',(-0.004136726,1.15025496390116E-19,8.88178419700125E-18));
#9865=CARTESIAN_POINT('Origin',(-0.004136726,1.15025496390116E-19,8.88178419700125E-18));
#9866=CARTESIAN_POINT('Origin',(0.00639999889435816,1.33725592594967E-10,
2.43522299685913E-19));
#9867=CARTESIAN_POINT('Origin',(0.00750000021337694,1.3831483908365E-10,
2.45725725091783E-19));
#9868=CARTESIAN_POINT('Origin',(0.0075,-1.31838984174237E-18,1.2490009027033E-18));
#9869=CARTESIAN_POINT('',(0.0075,-2.50440270425634E-18,0.02045));
#9870=CARTESIAN_POINT('Origin',(0.0075,0.,0.));
#9871=CARTESIAN_POINT('Origin',(4.25120033285821E-10,2.32696931299848E-18,
-2.53637255105429E-19));
#9872=CARTESIAN_POINT('',(-0.00413672599923392,-0.0130499999271107,-1.89332840771843E-18));
#9873=CARTESIAN_POINT('Origin',(4.25120034352053E-10,-0.01675,-2.30492064367725E-18));
#9874=CARTESIAN_POINT('',(-0.00413672599923392,-9.72427111671565E-12,0.0130499999635554));
#9875=CARTESIAN_POINT('Origin',(-0.00413672599923392,-2.48296911984889E-18,
-8.56610574398074E-20));
#9876=CARTESIAN_POINT('Origin',(-0.00413672599923392,-2.48296911984889E-18,
-8.56610574398074E-20));
#9877=CARTESIAN_POINT('Origin',(-0.0206375,0.,0.));
#9878=CARTESIAN_POINT('',(0.004136726,-0.02045,-1.97855791081413E-18));
#9879=CARTESIAN_POINT('',(0.004136726,-2.50440270425634E-18,0.02045));
#9880=CARTESIAN_POINT('Origin',(0.004136726,-1.49874617044541E-18,-8.88178419700125E-18));
#9881=CARTESIAN_POINT('Origin',(0.004136726,-1.49874617044541E-18,-8.88178419700125E-18));
#9882=CARTESIAN_POINT('',(-0.0206375,-2.50440270425634E-18,0.02045));
#9883=CARTESIAN_POINT('Origin',(-0.0206375,0.,0.));
#9884=CARTESIAN_POINT('',(-0.0075,-1.5981640728873E-18,0.01305));
#9885=CARTESIAN_POINT('',(-0.0206375,-1.5981640728873E-18,0.01305));
#9886=CARTESIAN_POINT('Origin',(-0.0075,0.,0.));
#9887=CARTESIAN_POINT('Origin',(-4.25120036303284E-10,3.75386134271222E-18,
6.07632462000188E-19));
#9888=CARTESIAN_POINT('',(0.00413672599923392,-2.67659699192252E-12,0.0130499999635553));
#9889=CARTESIAN_POINT('',(0.00413672599923392,-0.01305,-1.07231927942994E-18));
#9890=CARTESIAN_POINT('Origin',(0.00413672599923392,-3.3221160294436E-19,
2.22044604925031E-18));
#9891=CARTESIAN_POINT('Origin',(-4.25120034317525E-10,-0.01675,-1.44365092657163E-18));
#9892=CARTESIAN_POINT('Origin',(0.00413672599923392,-3.3221160294436E-19,
2.22044604925031E-18));
#9893=CARTESIAN_POINT('Origin',(-0.0075,-1.3010426069826E-19,-1.1666015375944E-18));
#9894=CARTESIAN_POINT('',(-0.00750000021337695,-7.32444758467801E-18,-0.00860000022986174));
#9895=CARTESIAN_POINT('',(-0.00750000021337695,-9.55563692214474E-13,0.00860000022983698));
#9896=CARTESIAN_POINT('Origin',(-0.00750000021337695,1.20438122996688E-10,
1.91155415755433E-19));
#9897=CARTESIAN_POINT('Origin',(-0.00750000021337695,-1.20438124044286E-10,
-1.263242268E-19));
#9898=CARTESIAN_POINT('Origin',(-0.0206375,0.,0.));
#9899=CARTESIAN_POINT('',(0.0075,-1.5981640728873E-18,0.01305));
#9900=CARTESIAN_POINT('Origin',(0.0075,0.,0.));
#9901=CARTESIAN_POINT('',(-0.0206375,-1.5981640728873E-18,0.01305));
#9902=CARTESIAN_POINT('Origin',(-0.00639999889435815,-1.33725589876008E-10,
-1.99489279445979E-19));
#9903=CARTESIAN_POINT('',(-0.00639999933187528,-1.78004529143068E-13,0.00749999975240887));
#9904=CARTESIAN_POINT('Origin',(-0.00639999889435815,-4.29138899262724E-13,
0.00860000107142784));
#9905=CARTESIAN_POINT('',(-0.00639999933187528,7.82593383085413E-14,-0.00749999975240887));
#9906=CARTESIAN_POINT('Origin',(-0.00639999977013826,-1.33725577217623E-10,
-2.22044604925031E-18));
#9907=CARTESIAN_POINT('Origin',(-0.00639999889435815,-4.29112928832131E-13,
-0.00860000107142784));
#9908=CARTESIAN_POINT('Origin',(-0.00639999889435816,1.33725589406987E-10,
2.62934110861178E-19));
#9909=CARTESIAN_POINT('Origin',(-0.00639999889435816,1.33725589406987E-10,
2.62934110861178E-19));
#9910=CARTESIAN_POINT('Origin',(0.0075,-1.3010426069826E-19,1.1666015375944E-18));
#9911=CARTESIAN_POINT('',(0.00750000021337695,-1.12844211802569E-18,0.00860000022986174));
#9912=CARTESIAN_POINT('',(0.00750000021337695,-9.55567354576375E-13,-0.00860000022983698));
#9913=CARTESIAN_POINT('Origin',(0.00750000021337695,1.20438122943562E-10,
-1.36910420000699E-19));
#9914=CARTESIAN_POINT('Origin',(0.00750000021337695,-1.20438123513651E-10,
2.9038238015475E-19));
#9915=CARTESIAN_POINT('Origin',(-0.0206375,0.,-2.49552314011156E-51));
#9916=CARTESIAN_POINT('',(0.00639999944717908,-3.41326938021997E-12,0.00749999987620436));
#9917=CARTESIAN_POINT('',(-0.0206375,-9.18485099360515E-19,0.0075));
#9918=CARTESIAN_POINT('',(0.00639999944670613,1.23481356905966E-13,-0.0074999998349392));
#9919=CARTESIAN_POINT('Origin',(0.0064,-1.93061231994698E-18,-5.55111512312578E-18));
#9920=CARTESIAN_POINT('Origin',(0.00639999889435815,1.33725588774518E-10,
-1.62015184442301E-19));
#9921=CARTESIAN_POINT('Origin',(0.00639999889435815,-1.33725589355705E-10,
3.07932432666985E-19));
#9922=CARTESIAN_POINT('Origin',(0.00639999889435815,-4.29128599184298E-13,
0.00860000107142785));
#9923=CARTESIAN_POINT('Origin',(0.00639999889435815,-4.2911240869608E-13,
-0.00860000107142785));
#9924=CARTESIAN_POINT('Origin',(0.00639999889435815,1.33725588774518E-10,
-1.62015184442301E-19));
#11042=UNCERTAINTY_MEASURE_WITH_UNIT(LENGTH_MEASURE(1.E-5),#11113,
'DISTANCE_ACCURACY_VALUE',
'Maximum model space distance between geometric entities at asserted c
onnectivities');
#11073=UNCERTAINTY_MEASURE_WITH_UNIT(LENGTH_MEASURE(1.E-5),#11113,
'DISTANCE_ACCURACY_VALUE',
'Maximum model space distance between geometric entities at asserted c
onnectivities');
#11081=(
GEOMETRIC_REPRESENTATION_CONTEXT(3)
GLOBAL_UNCERTAINTY_ASSIGNED_CONTEXT((#11042))
GLOBAL_UNIT_ASSIGNED_CONTEXT((#11113,#11114,#11115))
REPRESENTATION_CONTEXT('','3D')
);
#11112=(
GEOMETRIC_REPRESENTATION_CONTEXT(3)
GLOBAL_UNCERTAINTY_ASSIGNED_CONTEXT((#11073))
GLOBAL_UNIT_ASSIGNED_CONTEXT((#11113,#11114,#11115))
REPRESENTATION_CONTEXT('','3D')
);
#11113=(
LENGTH_UNIT()
NAMED_UNIT(*)
SI_UNIT($,.METRE.)
);
#11114=(
NAMED_UNIT(*)
PLANE_ANGLE_UNIT()
SI_UNIT($,.RADIAN.)
);
#11115=(
NAMED_UNIT(*)
SI_UNIT($,.STERADIAN.)
SOLID_ANGLE_UNIT()
);
#11123=SHAPE_DEFINITION_REPRESENTATION(#11161,#11236);
#11161=PRODUCT_DEFINITION_SHAPE('',$,#11275);
#11236=SHAPE_REPRESENTATION('',(#6679),#11081);
#11267=PRODUCT_DEFINITION_CONTEXT('part definition',#11383,'design');
#11275=PRODUCT_DEFINITION('Radial Ball Bearing 3',
'Radial Ball Bearing 3',#11313,#11267);
#11313=PRODUCT_DEFINITION_FORMATION('',$,#11392);
#11383=APPLICATION_CONTEXT(
'Core Data for Automotive Mechanical Design Process');
#11384=PRODUCT_CONTEXT('part definition',#11383,'mechanical');
#11392=PRODUCT('Radial Ball Bearing 3','Radial Ball Bearing 3',
'radial ball bearing_68_as_AS_ISO 15 RBB - 415 - 6,SI,NC,6_68__ DE    
10847',(#11384));
#11425=PRESENTATION_STYLE_ASSIGNMENT((#11429));
#11429=SURFACE_STYLE_USAGE(.BOTH.,#11433);
#11433=SURFACE_SIDE_STYLE('',(#11437));
#11437=SURFACE_STYLE_FILL_AREA(#11441);
#11441=FILL_AREA_STYLE('Opaque(255,242,232)',(#11445));
#11445=FILL_AREA_STYLE_COLOUR('Opaque(255,242,232)',#11449);
#11449=COLOUR_RGB('Opaque(255,242,232)',1.,0.949019607843137,0.909803921568627);
ENDSEC;
END-ISO-10303-21;
